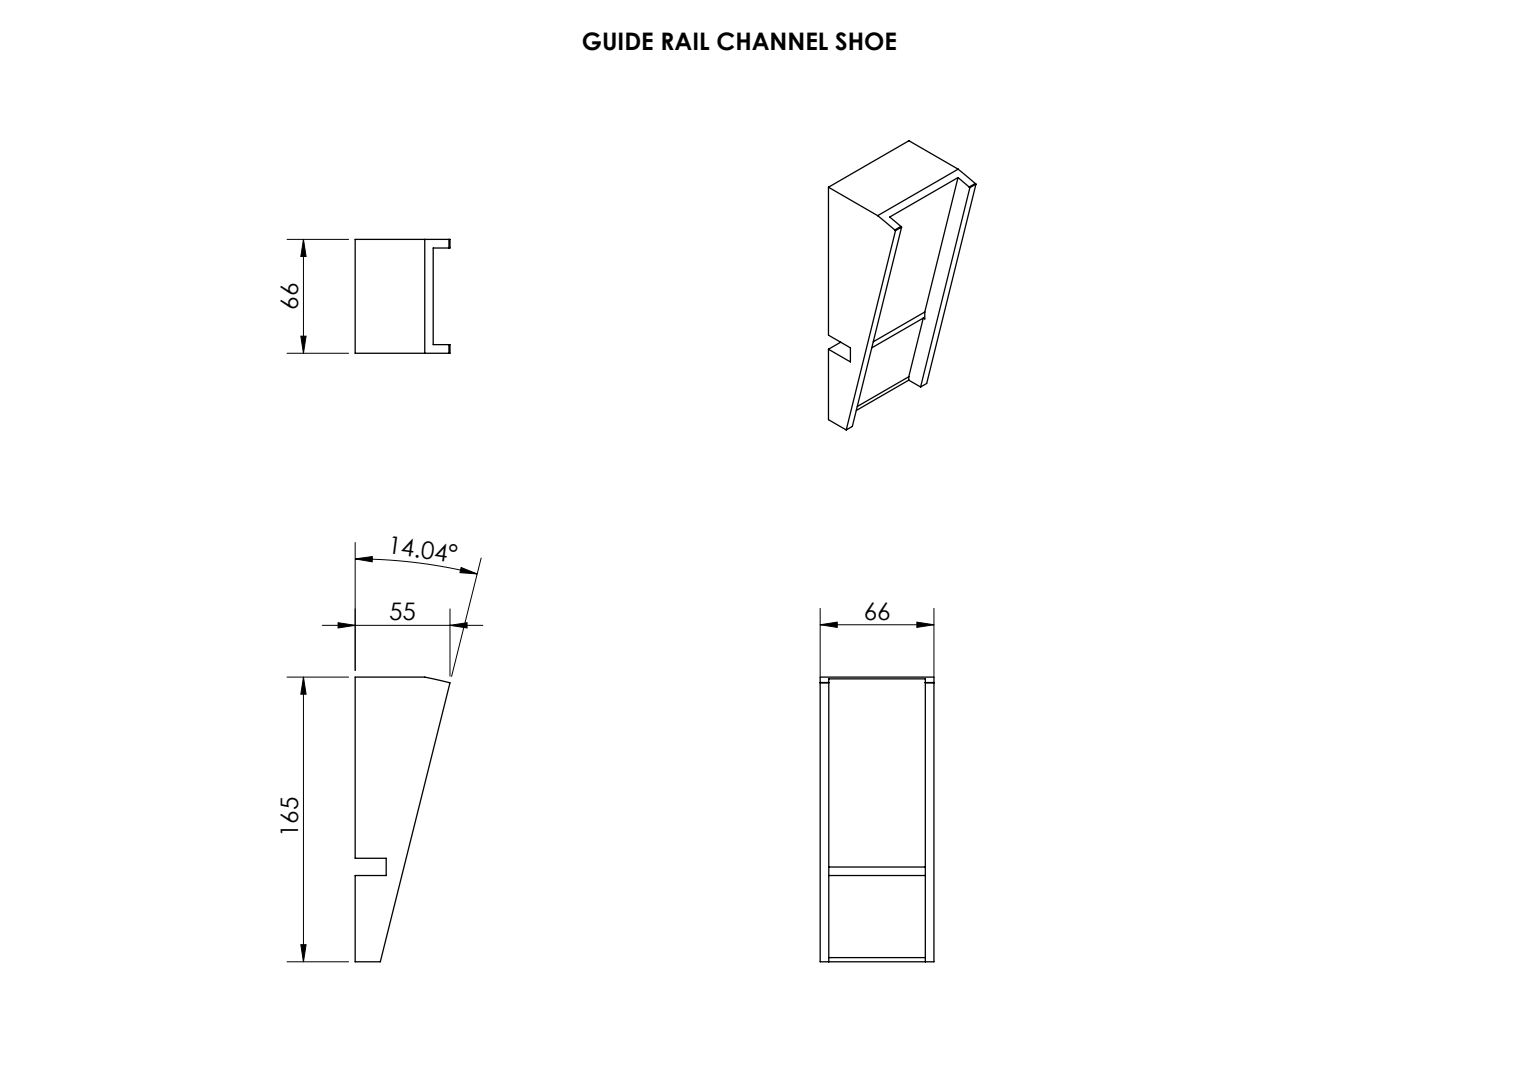
ISO-10303-21;
HEADER;
FILE_DESCRIPTION (('STEP AP214'),
    '1' );
FILE_NAME ('Guide Rail Channel Shoe.step',
    '2026-09-24T10:26:00',
    ( '' ),
    ( '' ),
    'SwSTEP 2.0',
    'SolidWorks 2026',
    '' );
FILE_SCHEMA (( 'AUTOMOTIVE_DESIGN' ));
ENDSEC;

DATA;
#6=CIRCLE ( 'NONE', #8168, 300.0000000000001137 ) ;
#19=DIRECTION ( 'NONE',  ( -0.2425356250363330801, 0.9701425001453319874, 0.000000000000000000 ) ) ;
#29=VERTEX_POINT ( 'NONE', #870 ) ;
#39=LINE ( 'NONE', #7923, #9383 ) ;
#42=( NAMED_UNIT ( * ) SI_UNIT ( $, .STERADIAN. ) SOLID_ANGLE_UNIT ( ) );
#81=ORIENTED_EDGE ( 'NONE', *, *, #3321, .F. ) ;
#100=ORIENTED_EDGE ( 'NONE', *, *, #751, .T. ) ;
#116=DIRECTION ( 'NONE',  ( 1.000000000000000000, 0.000000000000000000, 0.000000000000000000 ) ) ;
#118=EDGE_CURVE ( 'NONE', #4637, #7467, #9051, .T. ) ;
#154=CARTESIAN_POINT ( 'NONE',  ( 58.68170757442803165, 29.57655509336062849, -33.00000000000000000 ) ) ;
#162=DIRECTION ( 'NONE',  ( 0.000000000000000000, -1.000000000000000000, 0.000000000000000000 ) ) ;
#167=CARTESIAN_POINT ( 'NONE',  ( 0.000000000000000000, 0.000000000000000000, 0.000000000000000000 ) ) ;
#169=ORIENTED_EDGE ( 'NONE', *, *, #8329, .T. ) ;
#170=CARTESIAN_POINT ( 'NONE',  ( 59.91362529070399034, 29.57655509336063560, -28.00000000000000000 ) ) ;
#190=EDGE_LOOP ( 'NONE', ( #12989, #13833, #3490, #10771 ) ) ;
#193=PLANE ( 'NONE',  #1641 ) ;
#205=EDGE_CURVE ( 'NONE', #13026, #14419, #660, .T. ) ;
#259=FACE_OUTER_BOUND ( 'NONE', #5577, .T. ) ;
#285=COLOUR_RGB ( '', 0.40784314, 0.44705882, 0.49803922) ;
#310=DIRECTION ( 'NONE',  ( -0.000000000000000000, -0.000000000000000000, -1.000000000000000000 ) ) ;
#325=FILL_AREA_STYLE ('',( #4788 ) ) ;
#345=DIRECTION ( 'NONE',  ( 0.000000000000000000, 0.000000000000000000, -1.000000000000000000 ) ) ;
#366=DIRECTION ( 'NONE',  ( 0.000000000000000000, 0.000000000000000000, 1.000000000000000000 ) ) ;
#390=EDGE_CURVE ( 'NONE', #9890, #13868, #13175, .T. ) ;
#395=DIRECTION ( 'NONE',  ( 1.000000000000000000, 3.916739600140467622E-15, 0.000000000000000000 ) ) ;
#410=VECTOR ( 'NONE', #14385, 1000.000000000000000 ) ;
#431=ORIENTED_EDGE ( 'NONE', *, *, #13902, .F. ) ;
#449=ORIENTED_EDGE ( 'NONE', *, *, #10963, .T. ) ;
#469=CARTESIAN_POINT ( 'NONE',  ( 78.52142056027061301, -86.08568224108226730, -32.99999999999999289 ) ) ;
#487=( GEOMETRIC_REPRESENTATION_CONTEXT ( 3 ) GLOBAL_UNCERTAINTY_ASSIGNED_CONTEXT ( ( #2963 ) ) GLOBAL_UNIT_ASSIGNED_CONTEXT ( ( #1746, #1885, #3068 ) ) REPRESENTATION_CONTEXT ( 'NONE', 'WORKASPACE' ) );
#605=ORIENTED_EDGE ( 'NONE', *, *, #10788, .F. ) ;
#609=DIRECTION ( 'NONE',  ( 0.000000000000000000, -1.000000000000000000, 0.000000000000000000 ) ) ;
#650=LINE ( 'NONE', #12861, #14230 ) ;
#652=FILL_AREA_STYLE_COLOUR ( '', #8179 ) ;
#660=LINE ( 'NONE', #2704, #1726 ) ;
#670=DIRECTION ( 'NONE',  ( -3.916739600140467622E-15, 1.000000000000000000, 0.000000000000000000 ) ) ;
#687=VERTEX_POINT ( 'NONE', #13818 ) ;
#725=DIRECTION ( 'NONE',  ( 0.000000000000000000, -1.000000000000000000, 0.000000000000000000 ) ) ;
#733=DIRECTION ( 'NONE',  ( 0.2425356250363330801, -0.9701425001453319874, -0.000000000000000000 ) ) ;
#748=ORIENTED_EDGE ( 'NONE', *, *, #2973, .T. ) ;
#751=EDGE_CURVE ( 'NONE', #8097, #29, #10582, .T. ) ;
#754=ORIENTED_EDGE ( 'NONE', *, *, #2268, .T. ) ;
#757=ORIENTED_EDGE ( 'NONE', *, *, #2376, .F. ) ;
#758=( GEOMETRIC_REPRESENTATION_CONTEXT ( 3 ) GLOBAL_UNCERTAINTY_ASSIGNED_CONTEXT ( ( #7174 ) ) GLOBAL_UNIT_ASSIGNED_CONTEXT ( ( #1276, #6755, #8134 ) ) REPRESENTATION_CONTEXT ( 'NONE', 'WORKASPACE' ) );
#764=EDGE_LOOP ( 'NONE', ( #5468, #4866, #1029, #12657, #7119, #9076, #4306, #10621 ) ) ;
#774=VECTOR ( 'NONE', #10253, 1000.000000000000000 ) ;
#775=VECTOR ( 'NONE', #609, 1000.000000000000000 ) ;
#798=CARTESIAN_POINT ( 'NONE',  ( 76.68170757442801744, 39.57655509336063204, -33.00000000000000000 ) ) ;
#839=CARTESIAN_POINT ( 'NONE',  ( 31.38313257588132288, 143.6985259526512948, 28.00000000000000000 ) ) ;
#870=CARTESIAN_POINT ( 'NONE',  ( 76.68170757442804586, -20.42344490663941414, 33.00000000000000000 ) ) ;
#917=EDGE_CURVE ( 'NONE', #13885, #9506, #10868, .T. ) ;
#931=PRODUCT_CONTEXT ( 'NONE', #9027, 'mechanical' ) ;
#942=ORIENTED_EDGE ( 'NONE', *, *, #10788, .T. ) ;
#943=PLANE ( 'NONE',  #6123 ) ;
#944=EDGE_CURVE ( 'NONE', #7467, #1783, #14456, .T. ) ;
#954=AXIS2_PLACEMENT_3D ( 'NONE', #1864, #9695, #5154 ) ;
#1023=PRODUCT_DEFINITION_FORMATION_WITH_SPECIFIED_SOURCE ( 'ANY', '', #10212, .NOT_KNOWN. ) ;
#1029=ORIENTED_EDGE ( 'NONE', *, *, #14255, .T. ) ;
#1075=AXIS2_PLACEMENT_3D ( 'NONE', #6445, #8436, #7403 ) ;
#1183=VECTOR ( 'NONE', #14181, 1000.000000000000000 ) ;
#1190=VECTOR ( 'NONE', #3310, 1000.000000000000000 ) ;
#1215=DIRECTION ( 'NONE',  ( -0.2425356250363330801, 0.9701425001453319874, 0.000000000000000000 ) ) ;
#1216=EDGE_LOOP ( 'NONE', ( #3549, #605, #13304, #1795 ) ) ;
#1252=VECTOR ( 'NONE', #1971, 1000.000000000000000 ) ;
#1258=VECTOR ( 'NONE', #5303, 1000.000000000000000 ) ;
#1261=LINE ( 'NONE', #10450, #4207 ) ;
#1268=ORIENTED_EDGE ( 'NONE', *, *, #6526, .F. ) ;
#1276=( LENGTH_UNIT ( ) NAMED_UNIT ( * ) SI_UNIT ( .MILLI., .METRE. ) );
#1286=ORIENTED_EDGE ( 'NONE', *, *, #13904, .T. ) ;
#1342=DIRECTION ( 'NONE',  ( -1.000000000000000000, -1.927470528863119049E-16, 0.000000000000000000 ) ) ;
#1348=FACE_OUTER_BOUND ( 'NONE', #13937, .T. ) ;
#1358=LINE ( 'NONE', #5804, #6464 ) ;
#1366=DIRECTION ( 'NONE',  ( -1.000000000000000000, 0.000000000000000000, 0.000000000000000000 ) ) ;
#1376=CARTESIAN_POINT ( 'NONE',  ( 58.68170757442803165, 29.57655509336062849, -33.00000000000000000 ) ) ;
#1377=VERTEX_POINT ( 'NONE', #1649 ) ;
#1391=LINE ( 'NONE', #7911, #1671 ) ;
#1419=ORIENTED_EDGE ( 'NONE', *, *, #11341, .T. ) ;
#1502=ORIENTED_EDGE ( 'NONE', *, *, #3655, .T. ) ;
#1517=DIRECTION ( 'NONE',  ( 0.000000000000000000, 0.000000000000000000, 1.000000000000000000 ) ) ;
#1531=LINE ( 'NONE', #10681, #1666 ) ;
#1535=EDGE_CURVE ( 'NONE', #11633, #13672, #6590, .T. ) ;
#1586=FACE_OUTER_BOUND ( 'NONE', #7438, .T. ) ;
#1617=EDGE_CURVE ( 'NONE', #6928, #8393, #1391, .T. ) ;
#1637=ORIENTED_EDGE ( 'NONE', *, *, #13104, .T. ) ;
#1641=AXIS2_PLACEMENT_3D ( 'NONE', #5730, #345, #9335 ) ;
#1649=CARTESIAN_POINT ( 'NONE',  ( 22.28098402457126426, 141.4229888148237535, 33.00000000000000000 ) ) ;
#1664=CARTESIAN_POINT ( 'NONE',  ( 95.04167153547044222, -149.6197612287760705, 33.00000000000000000 ) ) ;
#1666=VECTOR ( 'NONE', #5975, 1000.000000000000000 ) ;
#1669=CARTESIAN_POINT ( 'NONE',  ( 76.68170757442804586, -20.42344490663941414, -33.00000000000000000 ) ) ;
#1671=VECTOR ( 'NONE', #310, 1000.000000000000000 ) ;
#1726=VECTOR ( 'NONE', #12961, 1000.000000000000000 ) ;
#1737=FACE_OUTER_BOUND ( 'NONE', #5106, .T. ) ;
#1746=( LENGTH_UNIT ( ) NAMED_UNIT ( * ) SI_UNIT ( .MILLI., .METRE. ) );
#1767=VERTEX_POINT ( 'NONE', #4988 ) ;
#1780=CARTESIAN_POINT ( 'NONE',  ( 78.52142056027061301, -86.08568224108226730, 28.00000000000000000 ) ) ;
#1783=VERTEX_POINT ( 'NONE', #7388 ) ;
#1784=UNCERTAINTY_MEASURE_WITH_UNIT (LENGTH_MEASURE( 1.000000000000000082E-05 ), #2241, 'distance_accuracy_value', 'NONE');
#1795=ORIENTED_EDGE ( 'NONE', *, *, #3657, .T. ) ;
#1814=ORIENTED_EDGE ( 'NONE', *, *, #7517, .T. ) ;
#1859=FACE_OUTER_BOUND ( 'NONE', #4265, .T. ) ;
#1863=ORIENTED_EDGE ( 'NONE', *, *, #8702, .F. ) ;
#1864=CARTESIAN_POINT ( 'NONE',  ( 36.31750732272606541, 144.5765550933605823, -199.4258611313499330 ) ) ;
#1885=( NAMED_UNIT ( * ) PLANE_ANGLE_UNIT ( ) SI_UNIT ( $, .RADIAN. ) );
#1923=AXIS2_PLACEMENT_3D ( 'NONE', #4562, #13481, #7898 ) ;
#1971=DIRECTION ( 'NONE',  ( 1.000000000000000000, 1.927470528863119049E-16, 0.000000000000000000 ) ) ;
#1973=PLANE ( 'NONE',  #10047 ) ;
#1995=DIRECTION ( 'NONE',  ( 1.000000000000000000, 0.000000000000000000, -3.576224061345501491E-16 ) ) ;
#2002=DIRECTION ( 'NONE',  ( -0.000000000000000000, -0.000000000000000000, -1.000000000000000000 ) ) ;
#2034=DIRECTION ( 'NONE',  ( 0.000000000000000000, 0.000000000000000000, -1.000000000000000000 ) ) ;
#2035=PLANE ( 'NONE',  #4449 ) ;
#2041=DIRECTION ( 'NONE',  ( 0.9701425001453325425, 0.2425356250363304988, 0.000000000000000000 ) ) ;
#2052=CARTESIAN_POINT ( 'NONE',  ( 71.80728622811317052, -20.42344490663941414, -27.99999999999999645 ) ) ;
#2080=ORIENTED_EDGE ( 'NONE', *, *, #12073, .T. ) ;
#2089=LINE ( 'NONE', #6752, #7978 ) ;
#2103=ORIENTED_EDGE ( 'NONE', *, *, #3418, .F. ) ;
#2109=FACE_OUTER_BOUND ( 'NONE', #10942, .T. ) ;
#2143=DIRECTION ( 'NONE',  ( 0.9701425001453319874, 0.2425356250363330801, 0.000000000000000000 ) ) ;
#2160=LINE ( 'NONE', #9912, #410 ) ;
#2164=AXIS2_PLACEMENT_3D ( 'NONE', #9423, #13830, #1366 ) ;
#2170=CARTESIAN_POINT ( 'NONE',  ( 59.91362529070399034, 29.57655509336062849, -28.00000000000000000 ) ) ;
#2171=DIRECTION ( 'NONE',  ( -3.916739600140467622E-15, 1.000000000000000000, 0.000000000000000000 ) ) ;
#2188=ORIENTED_EDGE ( 'NONE', *, *, #3988, .F. ) ;
#2219=CARTESIAN_POINT ( 'NONE',  ( 0.000000000000000000, -20.42344490663941414, -33.00000000000000000 ) ) ;
#2241=( LENGTH_UNIT ( ) NAMED_UNIT ( * ) SI_UNIT ( .MILLI., .METRE. ) );
#2245=ORIENTED_EDGE ( 'NONE', *, *, #6820, .F. ) ;
#2253=ADVANCED_FACE ( 'NONE', ( #2109 ), #2035, .F. ) ;
#2268=EDGE_CURVE ( 'NONE', #9459, #1783, #14266, .T. ) ;
#2272=FACE_OUTER_BOUND ( 'NONE', #2925, .T. ) ;
#2280=DIRECTION ( 'NONE',  ( -1.000000000000000000, 0.000000000000000000, 0.000000000000000000 ) ) ;
#2283=DIRECTION ( 'NONE',  ( -0.000000000000000000, -0.000000000000000000, -1.000000000000000000 ) ) ;
#2299=ORIENTED_EDGE ( 'NONE', *, *, #1535, .F. ) ;
#2316=VERTEX_POINT ( 'NONE', #8252 ) ;
#2362=VECTOR ( 'NONE', #9044, 1000.000000000000000 ) ;
#2367=VECTOR ( 'NONE', #2283, 1000.000000000000000 ) ;
#2376=EDGE_CURVE ( 'NONE', #9459, #11964, #1358, .T. ) ;
#2471=LINE ( 'NONE', #13614, #2362 ) ;
#2591=DIRECTION ( 'NONE',  ( 0.000000000000000000, 0.000000000000000000, 1.000000000000000000 ) ) ;
#2624=MECHANICAL_DESIGN_GEOMETRIC_PRESENTATION_REPRESENTATION('',(#10328),#11983);
#2671=CARTESIAN_POINT ( 'NONE',  ( 71.80728622811317052, -17.99808865627608512, -28.00000000000000000 ) ) ;
#2688=CARTESIAN_POINT ( 'NONE',  ( 76.68170757442804586, -20.42344490663941414, -199.4258611313499330 ) ) ;
#2691=ADVANCED_FACE ( 'NONE', ( #14116 ), #6465, .T. ) ;
#2692=FACE_OUTER_BOUND ( 'NONE', #4554, .T. ) ;
#2704=CARTESIAN_POINT ( 'NONE',  ( 76.68170757442801744, 144.5765550933605823, -199.4258611313499330 ) ) ;
#2837=VECTOR ( 'NONE', #366, 1000.000000000000000 ) ;
#2894=ORIENTED_EDGE ( 'NONE', *, *, #12073, .F. ) ;
#2925=EDGE_LOOP ( 'NONE', ( #10674, #14163, #9249, #8632, #13072, #942, #12028, #2103 ) ) ;
#2951=ORIENTED_EDGE ( 'NONE', *, *, #2973, .F. ) ;
#2958=VECTOR ( 'NONE', #3985, 999.9999999999998863 ) ;
#2963=UNCERTAINTY_MEASURE_WITH_UNIT (LENGTH_MEASURE( 1.000000000000000082E-05 ), #1746, 'distance_accuracy_value', 'NONE');
#2969=PLANE ( 'NONE',  #1075 ) ;
#2973=EDGE_CURVE ( 'NONE', #5297, #4637, #12601, .T. ) ;
#2992=DIRECTION ( 'NONE',  ( 1.000000000000000000, 3.916739600140467622E-15, 0.000000000000000000 ) ) ;
#3010=DIRECTION ( 'NONE',  ( -0.9701425001453325425, -0.2425356250363304988, 0.000000000000000000 ) ) ;
#3011=CARTESIAN_POINT ( 'NONE',  ( 62.10586122665989706, -20.42344490663939993, 33.00000000000000000 ) ) ;
#3060=DIRECTION ( 'NONE',  ( 1.000000000000000000, 0.000000000000000000, 0.000000000000000000 ) ) ;
#3068=( NAMED_UNIT ( * ) SI_UNIT ( $, .STERADIAN. ) SOLID_ANGLE_UNIT ( ) );
#3120=CARTESIAN_POINT ( 'NONE',  ( 88.22284556172391490, -83.66032599071898801, -28.00000000000000000 ) ) ;
#3144=EDGE_CURVE ( 'NONE', #5297, #4481, #12833, .T. ) ;
#3174=LINE ( 'NONE', #2219, #6591 ) ;
#3310=DIRECTION ( 'NONE',  ( 1.000000000000000000, 0.000000000000000000, 0.000000000000000000 ) ) ;
#3318=VECTOR ( 'NONE', #670, 1000.000000000000000 ) ;
#3321=EDGE_CURVE ( 'NONE', #6195, #10355, #8937, .T. ) ;
#3340=CARTESIAN_POINT ( 'NONE',  ( 22.28098402457129268, 141.4229888148237251, 28.00000000000000000 ) ) ;
#3343=ORIENTED_EDGE ( 'NONE', *, *, #944, .F. ) ;
#3345=DIRECTION ( 'NONE',  ( 0.000000000000000000, 0.000000000000000000, 1.000000000000000000 ) ) ;
#3359=ORIENTED_EDGE ( 'NONE', *, *, #5495, .T. ) ;
#3402=EDGE_CURVE ( 'NONE', #13672, #4341, #11854, .T. ) ;
#3418=EDGE_CURVE ( 'NONE', #1767, #6248, #10583, .T. ) ;
#3448=DIRECTION ( 'NONE',  ( -1.000000000000000000, 0.000000000000000000, 0.000000000000000000 ) ) ;
#3487=( NAMED_UNIT ( * ) PLANE_ANGLE_UNIT ( ) SI_UNIT ( $, .RADIAN. ) );
#3490=ORIENTED_EDGE ( 'NONE', *, *, #5495, .F. ) ;
#3533=VECTOR ( 'NONE', #10987, 1000.000000000000000 ) ;
#3541=ADVANCED_FACE ( 'NONE', ( #1737 ), #9841, .T. ) ;
#3542=VECTOR ( 'NONE', #3817, 1000.000000000000000 ) ;
#3549=ORIENTED_EDGE ( 'NONE', *, *, #9120, .T. ) ;
#3622=EDGE_CURVE ( 'NONE', #6997, #10870, #2089, .T. ) ;
#3627=CARTESIAN_POINT ( 'NONE',  ( 76.68170757442796059, 3.003422806631532356E-13, -199.4258611313499330 ) ) ;
#3638=CIRCLE ( 'NONE', #12999, 300.0000000000001137 ) ;
#3642=VERTEX_POINT ( 'NONE', #8877 ) ;
#3655=EDGE_CURVE ( 'NONE', #4481, #7467, #6833, .T. ) ;
#3657=EDGE_CURVE ( 'NONE', #5508, #3642, #39, .T. ) ;
#3662=LINE ( 'NONE', #8098, #8406 ) ;
#3722=LINE ( 'NONE', #6781, #7013 ) ;
#3757=LINE ( 'NONE', #11573, #12946 ) ;
#3817=DIRECTION ( 'NONE',  ( -1.000000000000000000, 0.000000000000000000, 0.000000000000000000 ) ) ;
#3901=EDGE_CURVE ( 'NONE', #4341, #6772, #14016, .T. ) ;
#3912=FACE_OUTER_BOUND ( 'NONE', #190, .T. ) ;
#3916=VECTOR ( 'NONE', #1215, 999.9999999999998863 ) ;
#3981=AXIS2_PLACEMENT_3D ( 'NONE', #8549, #9580, #3010 ) ;
#3985=DIRECTION ( 'NONE',  ( -0.9701425001453319874, -0.2425356250363330801, -0.000000000000000000 ) ) ;
#3988=EDGE_CURVE ( 'NONE', #1377, #11964, #7544, .T. ) ;
#4054=CARTESIAN_POINT ( 'NONE',  ( 58.68170757442803165, -86.08568224108226730, -28.00000000000000000 ) ) ;
#4068=ORIENTED_EDGE ( 'NONE', *, *, #10686, .T. ) ;
#4128=VERTEX_POINT ( 'NONE', #14373 ) ;
#4158=ORIENTED_EDGE ( 'NONE', *, *, #12918, .T. ) ;
#4207=VECTOR ( 'NONE', #162, 1000.000000000000000 ) ;
#4265=EDGE_LOOP ( 'NONE', ( #2188, #13222, #7506, #10107 ) ) ;
#4270=VECTOR ( 'NONE', #8995, 999.9999999999998863 ) ;
#4306=ORIENTED_EDGE ( 'NONE', *, *, #390, .T. ) ;
#4319=CARTESIAN_POINT ( 'NONE',  ( 88.22284556172391490, -83.66032599071898801, 28.00000000000000000 ) ) ;
#4341=VERTEX_POINT ( 'NONE', #11796 ) ;
#4345=CARTESIAN_POINT ( 'NONE',  ( 36.31750732272606541, 144.5765550933605823, 33.00000000000000000 ) ) ;
#4352=EDGE_CURVE ( 'NONE', #13229, #9890, #8564, .T. ) ;
#4353=FACE_OUTER_BOUND ( 'NONE', #9545, .T. ) ;
#4361=EDGE_CURVE ( 'NONE', #1377, #13885, #6147, .T. ) ;
#4362=CARTESIAN_POINT ( 'NONE',  ( 58.68170757442803165, 29.57655509336062849, -28.00000000000000000 ) ) ;
#4387=ORIENTED_EDGE ( 'NONE', *, *, #944, .T. ) ;
#4437=LINE ( 'NONE', #8794, #3533 ) ;
#4449=AXIS2_PLACEMENT_3D ( 'NONE', #5324, #13310, #8550 ) ;
#4481=VERTEX_POINT ( 'NONE', #2052 ) ;
#4483=VECTOR ( 'NONE', #1342, 1000.000000000000000 ) ;
#4488=ADVANCED_FACE ( 'NONE', ( #2272 ), #943, .F. ) ;
#4536=ORIENTED_EDGE ( 'NONE', *, *, #9120, .F. ) ;
#4554=EDGE_LOOP ( 'NONE', ( #11599, #8685, #6383, #1863, #11350, #2894, #13470, #4387, #4158 ) ) ;
#4561=ADVANCED_BREP_SHAPE_REPRESENTATION ( '', ( #11635, #11025 ), #758 ) ;
#4562=CARTESIAN_POINT ( 'NONE',  ( 76.68170757442801744, 29.57655509336063204, -33.00000000000000000 ) ) ;
#4618=CARTESIAN_POINT ( 'NONE',  ( 58.68170757442803165, 39.57655509336063204, -33.00000000000000000 ) ) ;
#4637=VERTEX_POINT ( 'NONE', #7003 ) ;
#4640=EDGE_LOOP ( 'NONE', ( #8368, #1419, #13334, #100, #2245, #754, #3343, #7325 ) ) ;
#4644=VECTOR ( 'NONE', #12554, 1000.000000000000000 ) ;
#4655=ORIENTED_EDGE ( 'NONE', *, *, #3657, .F. ) ;
#4719=SURFACE_SIDE_STYLE ('',( #12473 ) ) ;
#4731=VERTEX_POINT ( 'NONE', #7629 ) ;
#4732=CARTESIAN_POINT ( 'NONE',  ( 31.41872415839353039, 143.5561596226025074, -28.00000000000000000 ) ) ;
#4733=ORIENTED_EDGE ( 'NONE', *, *, #10431, .F. ) ;
#4734=ORIENTED_EDGE ( 'NONE', *, *, #390, .F. ) ;
#4744=ORIENTED_EDGE ( 'NONE', *, *, #1617, .T. ) ;
#4788=FILL_AREA_STYLE_COLOUR ( '', #285 ) ;
#4831=VECTOR ( 'NONE', #11737, 1000.000000000000000 ) ;
#4832=EDGE_LOOP ( 'NONE', ( #9169, #12336, #14242, #4068 ) ) ;
#4866=ORIENTED_EDGE ( 'NONE', *, *, #3418, .T. ) ;
#4918=CARTESIAN_POINT ( 'NONE',  ( 21.68170757442799967, 141.2731697022880155, -28.00000000000000000 ) ) ;
#4934=CARTESIAN_POINT ( 'NONE',  ( 21.68170757442799967, 141.2731697022880155, -32.99999999999999289 ) ) ;
#4951=AXIS2_PLACEMENT_3D ( 'NONE', #10869, #8532, #3060 ) ;
#4953=EDGE_CURVE ( 'NONE', #13868, #9429, #7712, .T. ) ;
#4985=ORIENTED_EDGE ( 'NONE', *, *, #205, .T. ) ;
#4988=CARTESIAN_POINT ( 'NONE',  ( 58.68170757442803165, 29.57655509336062849, 27.99999999999999645 ) ) ;
#5026=LINE ( 'NONE', #5170, #1183 ) ;
#5027=EDGE_CURVE ( 'NONE', #8393, #11633, #3638, .T. ) ;
#5055=DIRECTION ( 'NONE',  ( -0.000000000000000000, -0.000000000000000000, -1.000000000000000000 ) ) ;
#5082=ADVANCED_FACE ( 'NONE', ( #3912 ), #8061, .T. ) ;
#5104=ORIENTED_EDGE ( 'NONE', *, *, #2376, .T. ) ;
#5106=EDGE_LOOP ( 'NONE', ( #11663, #6184, #10149, #7042, #11543, #2299, #7476, #9228 ) ) ;
#5135=DIRECTION ( 'NONE',  ( -0.2425356250363330801, 0.9701425001453319874, 0.000000000000000000 ) ) ;
#5145=ORIENTED_EDGE ( 'NONE', *, *, #6298, .T. ) ;
#5154=DIRECTION ( 'NONE',  ( 0.000000000000000000, 0.000000000000000000, -1.000000000000000000 ) ) ;
#5170=CARTESIAN_POINT ( 'NONE',  ( 76.68170757442801744, 39.57655509336063204, -33.00000000000000000 ) ) ;
#5172=ADVANCED_FACE ( 'NONE', ( #1859 ), #2969, .F. ) ;
#5190=LINE ( 'NONE', #12970, #9623 ) ;
#5195=VECTOR ( 'NONE', #11598, 1000.000000000000000 ) ;
#5292=EDGE_LOOP ( 'NONE', ( #12843, #7817, #748, #2080 ) ) ;
#5294=LINE ( 'NONE', #3120, #12559 ) ;
#5295=EDGE_CURVE ( 'NONE', #13026, #5508, #3662, .T. ) ;
#5297=VERTEX_POINT ( 'NONE', #11472 ) ;
#5303=DIRECTION ( 'NONE',  ( -0.9701425001453325425, -0.2425356250363304988, 0.000000000000000000 ) ) ;
#5323=CARTESIAN_POINT ( 'NONE',  ( 76.68170757442796059, 3.003422806631532356E-13, 33.00000000000000000 ) ) ;
#5324=CARTESIAN_POINT ( 'NONE',  ( 78.52142056027061301, -86.08568224108226730, -28.00000000000000000 ) ) ;
#5391=CARTESIAN_POINT ( 'NONE',  ( 78.52142056027055617, 29.57655509336062849, -28.00000000000000000 ) ) ;
#5417=PLANE ( 'NONE',  #1923 ) ;
#5429=ADVANCED_FACE ( 'NONE', ( #8481 ), #7374, .F. ) ;
#5441=DIRECTION ( 'NONE',  ( 1.000000000000000000, 0.000000000000000000, 0.000000000000000000 ) ) ;
#5466=EDGE_CURVE ( 'NONE', #13885, #6928, #6, .T. ) ;
#5468=ORIENTED_EDGE ( 'NONE', *, *, #11730, .T. ) ;
#5492=LINE ( 'NONE', #9961, #4270 ) ;
#5495=EDGE_CURVE ( 'NONE', #29, #687, #7507, .T. ) ;
#5498=PLANE ( 'NONE',  #13650 ) ;
#5500=ADVANCED_FACE ( 'NONE', ( #13102 ), #1973, .T. ) ;
#5507=ORIENTED_EDGE ( 'NONE', *, *, #5027, .T. ) ;
#5508=VERTEX_POINT ( 'NONE', #798 ) ;
#5518=CARTESIAN_POINT ( 'NONE',  ( 71.80728622811317052, -20.42344490663941414, 28.00000000000000000 ) ) ;
#5528=AXIS2_PLACEMENT_3D ( 'NONE', #12031, #2002, #13351 ) ;
#5538=LINE ( 'NONE', #10010, #6079 ) ;
#5577=EDGE_LOOP ( 'NONE', ( #1286, #5507, #8075, #7936, #12667, #10442, #1814, #4734, #12975 ) ) ;
#5635=CARTESIAN_POINT ( 'NONE',  ( 22.28098402457126426, 141.4229888148238103, 1.219362754841566419E-12 ) ) ;
#5653=FACE_OUTER_BOUND ( 'NONE', #8593, .T. ) ;
#5654=CARTESIAN_POINT ( 'NONE',  ( 95.04167153547044222, -149.6197612287760705, -28.00000000000000000 ) ) ;
#5694=LINE ( 'NONE', #154, #9376 ) ;
#5730=CARTESIAN_POINT ( 'NONE',  ( 88.22284556172391490, -83.66032599071898801, 28.00000000000000000 ) ) ;
#5768=ADVANCED_FACE ( 'NONE', ( #2692 ), #193, .T. ) ;
#5793=ORIENTED_EDGE ( 'NONE', *, *, #3321, .T. ) ;
#5794=PLANE ( 'NONE',  #11865 ) ;
#5804=CARTESIAN_POINT ( 'NONE',  ( 78.52142056027061301, -86.08568224108226730, 33.00000000000000000 ) ) ;
#5849=EDGE_CURVE ( 'NONE', #5508, #6997, #5026, .T. ) ;
#5870=DIRECTION ( 'NONE',  ( 1.000000000000000000, 0.000000000000000000, 0.000000000000000000 ) ) ;
#5886=LINE ( 'NONE', #11384, #4644 ) ;
#5897=ORIENTED_EDGE ( 'NONE', *, *, #3402, .T. ) ;
#5938=CARTESIAN_POINT ( 'NONE',  ( 78.52142056027061301, -86.08568224108226730, -28.00000000000000000 ) ) ;
#5958=CARTESIAN_POINT ( 'NONE',  ( 59.91362529070399034, 29.57655509336062849, 28.00000000000000000 ) ) ;
#5975=DIRECTION ( 'NONE',  ( 0.000000000000000000, 0.000000000000000000, -1.000000000000000000 ) ) ;
#5983=VECTOR ( 'NONE', #2591, 1000.000000000000000 ) ;
#5993=ADVANCED_FACE ( 'NONE', ( #5653 ), #11578, .F. ) ;
#5999=PRODUCT_DEFINITION_SHAPE ( 'NONE', 'NONE',  #12500 ) ;
#6047=ORIENTED_EDGE ( 'NONE', *, *, #5295, .T. ) ;
#6055=LINE ( 'NONE', #13630, #3542 ) ;
#6079=VECTOR ( 'NONE', #2041, 1000.000000000000000 ) ;
#6101=ORIENTED_EDGE ( 'NONE', *, *, #10400, .T. ) ;
#6113=DIRECTION ( 'NONE',  ( -0.000000000000000000, -0.000000000000000000, 1.000000000000000000 ) ) ;
#6123=AXIS2_PLACEMENT_3D ( 'NONE', #10094, #3448, #14356 ) ;
#6139=AXIS2_PLACEMENT_3D ( 'NONE', #7558, #6250, #8449 ) ;
#6146=VECTOR ( 'NONE', #13427, 1000.000000000000000 ) ;
#6147=LINE ( 'NONE', #14214, #11993 ) ;
#6184=ORIENTED_EDGE ( 'NONE', *, *, #4361, .F. ) ;
#6195=VERTEX_POINT ( 'NONE', #10784 ) ;
#6196=CARTESIAN_POINT ( 'NONE',  ( 22.28098402457126426, 141.4229888148238103, -28.00000000000000000 ) ) ;
#6248=VERTEX_POINT ( 'NONE', #14444 ) ;
#6250=DIRECTION ( 'NONE',  ( -0.9701425001453319874, -0.2425356250363330801, 0.000000000000000000 ) ) ;
#6280=LINE ( 'NONE', #9725, #3318 ) ;
#6298=EDGE_CURVE ( 'NONE', #10870, #2316, #4437, .T. ) ;
#6302=ORIENTED_EDGE ( 'NONE', *, *, #10686, .F. ) ;
#6352=DIRECTION ( 'NONE',  ( 0.000000000000000000, 1.000000000000000000, 0.000000000000000000 ) ) ;
#6382=CARTESIAN_POINT ( 'NONE',  ( 71.80728622811317052, 38.49793223363091954, -28.00000000000000000 ) ) ;
#6383=ORIENTED_EDGE ( 'NONE', *, *, #8329, .F. ) ;
#6394=ORIENTED_EDGE ( 'NONE', *, *, #3988, .T. ) ;
#6425=ORIENTED_EDGE ( 'NONE', *, *, #5849, .T. ) ;
#6445=CARTESIAN_POINT ( 'NONE',  ( -31.96535124910143821, 127.8614049964057813, 1.219362754841566419E-12 ) ) ;
#6464=VECTOR ( 'NONE', #12491, 999.9999999999998863 ) ;
#6465=PLANE ( 'NONE',  #14233 ) ;
#6508=CARTESIAN_POINT ( 'NONE',  ( 62.10586122665986863, -20.42344490663941414, -27.99999999999999645 ) ) ;
#6524=DIRECTION ( 'NONE',  ( 0.000000000000000000, 0.000000000000000000, 1.000000000000000000 ) ) ;
#6526=EDGE_CURVE ( 'NONE', #10492, #6248, #1261, .T. ) ;
#6590=LINE ( 'NONE', #5635, #2367 ) ;
#6591=VECTOR ( 'NONE', #2280, 1000.000000000000000 ) ;
#6622=LINE ( 'NONE', #4319, #3916 ) ;
#6659=LINE ( 'NONE', #6508, #8116 ) ;
#6737=LINE ( 'NONE', #14368, #6146 ) ;
#6739=PRODUCT_DEFINITION_CONTEXT ( 'detailed design', #10449, 'design' ) ;
#6752=CARTESIAN_POINT ( 'NONE',  ( 58.68170757442803165, 39.57655509336063204, -33.00000000000000000 ) ) ;
#6755=( NAMED_UNIT ( * ) PLANE_ANGLE_UNIT ( ) SI_UNIT ( $, .RADIAN. ) );
#6772=VERTEX_POINT ( 'NONE', #11602 ) ;
#6781=CARTESIAN_POINT ( 'NONE',  ( 76.68170757442796059, 3.003422806631532356E-13, -33.00000000000000000 ) ) ;
#6789=DIRECTION ( 'NONE',  ( 0.000000000000000000, -1.000000000000000000, 0.000000000000000000 ) ) ;
#6820=EDGE_CURVE ( 'NONE', #9459, #29, #5886, .T. ) ;
#6833=LINE ( 'NONE', #11299, #12432 ) ;
#6928=VERTEX_POINT ( 'NONE', #13411 ) ;
#6990=CARTESIAN_POINT ( 'NONE',  ( 21.68170757442799967, 141.2731697022880155, -32.99999999999999289 ) ) ;
#6997=VERTEX_POINT ( 'NONE', #11092 ) ;
#7003=CARTESIAN_POINT ( 'NONE',  ( 71.80728622811317052, -17.99808865627608512, 28.00000000000000000 ) ) ;
#7011=CARTESIAN_POINT ( 'NONE',  ( 58.68170757442803165, 34.50422595846453078, -28.00000000000000000 ) ) ;
#7013=VECTOR ( 'NONE', #7878, 1000.000000000000000 ) ;
#7042=ORIENTED_EDGE ( 'NONE', *, *, #3901, .F. ) ;
#7119=ORIENTED_EDGE ( 'NONE', *, *, #6298, .F. ) ;
#7121=FACE_OUTER_BOUND ( 'NONE', #7956, .T. ) ;
#7127=DIRECTION ( 'NONE',  ( 0.000000000000000000, 0.000000000000000000, 1.000000000000000000 ) ) ;
#7128=CARTESIAN_POINT ( 'NONE',  ( 58.68170757442803165, 29.57655509336062849, -33.00000000000000000 ) ) ;
#7171=DIRECTION ( 'NONE',  ( -0.2425356250363330801, 0.9701425001453319874, 0.000000000000000000 ) ) ;
#7174=UNCERTAINTY_MEASURE_WITH_UNIT (LENGTH_MEASURE( 1.000000000000000082E-05 ), #1276, 'distance_accuracy_value', 'NONE');
#7190=LINE ( 'NONE', #4934, #10247 ) ;
#7298=EDGE_CURVE ( 'NONE', #10355, #13672, #7190, .T. ) ;
#7304=ORIENTED_EDGE ( 'NONE', *, *, #12918, .F. ) ;
#7310=PLANE ( 'NONE',  #8448 ) ;
#7325=ORIENTED_EDGE ( 'NONE', *, *, #3655, .F. ) ;
#7344=FACE_OUTER_BOUND ( 'NONE', #4832, .T. ) ;
#7374=PLANE ( 'NONE',  #3981 ) ;
#7388=CARTESIAN_POINT ( 'NONE',  ( 62.10586122665986863, -20.42344490663941414, 28.00000000000000000 ) ) ;
#7389=SHAPE_REPRESENTATION ( 'Guide Rail Channel Shoe', ( #11025 ), #758 ) ;
#7403=DIRECTION ( 'NONE',  ( -0.9701425001453325425, -0.2425356250363304988, 0.000000000000000000 ) ) ;
#7413=PLANE ( 'NONE',  #6139 ) ;
#7426=PRESENTATION_STYLE_ASSIGNMENT (( #9639 ) ) ;
#7438=EDGE_LOOP ( 'NONE', ( #6302, #8058, #6394, #757, #11181, #3359, #11732, #1268, #4536, #9883 ) ) ;
#7467=VERTEX_POINT ( 'NONE', #11078 ) ;
#7476=ORIENTED_EDGE ( 'NONE', *, *, #5027, .F. ) ;
#7506=ORIENTED_EDGE ( 'NONE', *, *, #917, .T. ) ;
#7507=LINE ( 'NONE', #5323, #11678 ) ;
#7508=VECTOR ( 'NONE', #5135, 999.9999999999998863 ) ;
#7510=DIRECTION ( 'NONE',  ( 0.000000000000000000, 0.000000000000000000, -1.000000000000000000 ) ) ;
#7512=CARTESIAN_POINT ( 'NONE',  ( 76.68170757442801744, 39.57655509336063204, 33.00000000000000000 ) ) ;
#7513=FACE_OUTER_BOUND ( 'NONE', #1216, .T. ) ;
#7517=EDGE_CURVE ( 'NONE', #5297, #13868, #5294, .T. ) ;
#7544=LINE ( 'NONE', #11810, #2958 ) ;
#7555=VECTOR ( 'NONE', #8056, 1000.000000000000000 ) ;
#7558=CARTESIAN_POINT ( 'NONE',  ( 88.22284556172391490, -83.66032599071898801, -28.00000000000000000 ) ) ;
#7629=CARTESIAN_POINT ( 'NONE',  ( 58.68170757442803165, 34.50422595846454499, 28.00000000000000000 ) ) ;
#7712=LINE ( 'NONE', #2170, #12809 ) ;
#7757=DIRECTION ( 'NONE',  ( 0.000000000000000000, 0.000000000000000000, 1.000000000000000000 ) ) ;
#7817=ORIENTED_EDGE ( 'NONE', *, *, #7517, .F. ) ;
#7843=DIRECTION ( 'NONE',  ( -0.2425356250363330801, 0.9701425001453319874, 0.000000000000000000 ) ) ;
#7846=VERTEX_POINT ( 'NONE', #10772 ) ;
#7878=DIRECTION ( 'NONE',  ( 3.916739600140467622E-15, -1.000000000000000000, -0.000000000000000000 ) ) ;
#7898=DIRECTION ( 'NONE',  ( 1.000000000000000000, 1.927470528863118802E-16, 0.000000000000000000 ) ) ;
#7911=CARTESIAN_POINT ( 'NONE',  ( 31.41872415839353039, 143.5561596226024790, 28.00000000000000000 ) ) ;
#7923=CARTESIAN_POINT ( 'NONE',  ( 76.68170757442801744, 39.57655509336063204, -33.00000000000000000 ) ) ;
#7934=EDGE_CURVE ( 'NONE', #4128, #4481, #6659, .T. ) ;
#7936=ORIENTED_EDGE ( 'NONE', *, *, #9847, .F. ) ;
#7955=CARTESIAN_POINT ( 'NONE',  ( 71.80728622811317052, 38.49793223363091954, 28.00000000000000000 ) ) ;
#7956=EDGE_LOOP ( 'NONE', ( #169, #4744, #12317, #4733 ) ) ;
#7978=VECTOR ( 'NONE', #13374, 1000.000000000000000 ) ;
#8056=DIRECTION ( 'NONE',  ( -1.000000000000000000, 0.000000000000000000, -3.576224061345501491E-16 ) ) ;
#8058=ORIENTED_EDGE ( 'NONE', *, *, #10577, .T. ) ;
#8061=PLANE ( 'NONE',  #10645 ) ;
#8075=ORIENTED_EDGE ( 'NONE', *, *, #10303, .F. ) ;
#8090=ORIENTED_EDGE ( 'NONE', *, *, #2268, .F. ) ;
#8097=VERTEX_POINT ( 'NONE', #1669 ) ;
#8098=CARTESIAN_POINT ( 'NONE',  ( 76.68170757442796059, 3.003422806631532356E-13, -33.00000000000000000 ) ) ;
#8116=VECTOR ( 'NONE', #1995, 1000.000000000000000 ) ;
#8134=( NAMED_UNIT ( * ) SI_UNIT ( $, .STERADIAN. ) SOLID_ANGLE_UNIT ( ) );
#8168=AXIS2_PLACEMENT_3D ( 'NONE', #10749, #12064, #11850 ) ;
#8179=COLOUR_RGB ( '', 0.40784314, 0.44705882, 0.49803922) ;
#8189=ORIENTED_EDGE ( 'NONE', *, *, #9847, .T. ) ;
#8190=CIRCLE ( 'NONE', #13356, 300.0000000000001137 ) ;
#8220=ORIENTED_EDGE ( 'NONE', *, *, #11206, .F. ) ;
#8252=CARTESIAN_POINT ( 'NONE',  ( 76.68170757442801744, 29.57655509336063204, -33.00000000000000000 ) ) ;
#8290=DIRECTION ( 'NONE',  ( 0.000000000000000000, 0.000000000000000000, 1.000000000000000000 ) ) ;
#8329=EDGE_CURVE ( 'NONE', #4731, #6928, #6622, .T. ) ;
#8351=CARTESIAN_POINT ( 'NONE',  ( 36.31750732272606541, 144.5765550933605823, -199.4258611313499330 ) ) ;
#8357=DIRECTION ( 'NONE',  ( -3.916739600140467622E-15, 1.000000000000000000, 0.000000000000000000 ) ) ;
#8367=DIRECTION ( 'NONE',  ( 1.000000000000000000, 0.000000000000000000, 0.000000000000000000 ) ) ;
#8368=ORIENTED_EDGE ( 'NONE', *, *, #7934, .F. ) ;
#8393=VERTEX_POINT ( 'NONE', #4732 ) ;
#8401=DIRECTION ( 'NONE',  ( 0.000000000000000000, 0.000000000000000000, -1.000000000000000000 ) ) ;
#8406=VECTOR ( 'NONE', #13626, 1000.000000000000000 ) ;
#8436=DIRECTION ( 'NONE',  ( 0.2425356250363304988, -0.9701425001453325425, -0.000000000000000000 ) ) ;
#8448=AXIS2_PLACEMENT_3D ( 'NONE', #12001, #6352, #10829 ) ;
#8449=DIRECTION ( 'NONE',  ( 0.2425356250363330801, -0.9701425001453319874, -0.000000000000000000 ) ) ;
#8475=ADVANCED_FACE ( 'NONE', ( #1348 ), #5794, .F. ) ;
#8481=FACE_OUTER_BOUND ( 'NONE', #11329, .T. ) ;
#8532=DIRECTION ( 'NONE',  ( 0.000000000000000000, 0.000000000000000000, 1.000000000000000000 ) ) ;
#8549=CARTESIAN_POINT ( 'NONE',  ( -31.96535124910143821, 127.8614049964057813, 1.219362754841566419E-12 ) ) ;
#8550=DIRECTION ( 'NONE',  ( -0.2425356250363330801, 0.9701425001453319874, 0.000000000000000000 ) ) ;
#8564=LINE ( 'NONE', #4054, #775 ) ;
#8593=EDGE_LOOP ( 'NONE', ( #12591, #5897, #12415, #6047, #6425, #12852, #5145, #6101, #1637, #5793 ) ) ;
#8632=ORIENTED_EDGE ( 'NONE', *, *, #11989, .F. ) ;
#8685=ORIENTED_EDGE ( 'NONE', *, *, #5466, .T. ) ;
#8702=EDGE_CURVE ( 'NONE', #1767, #4731, #2160, .T. ) ;
#8788=CARTESIAN_POINT ( 'NONE',  ( 78.52142056027061301, -86.08568224108226730, 33.00000000000000000 ) ) ;
#8794=CARTESIAN_POINT ( 'NONE',  ( 76.68170757442801744, 29.57655509336063204, -33.00000000000000000 ) ) ;
#8877=CARTESIAN_POINT ( 'NONE',  ( 76.68170757442801744, 39.57655509336063204, 33.00000000000000000 ) ) ;
#8903=LINE ( 'NONE', #7512, #13753 ) ;
#8937=LINE ( 'NONE', #9820, #12531 ) ;
#8995=DIRECTION ( 'NONE',  ( -0.2425356250363330801, 0.9701425001453319874, 0.000000000000000000 ) ) ;
#9000=ORIENTED_EDGE ( 'NONE', *, *, #7298, .F. ) ;
#9027=APPLICATION_CONTEXT ( 'automotive_design' ) ;
#9044=DIRECTION ( 'NONE',  ( 0.000000000000000000, 0.000000000000000000, -1.000000000000000000 ) ) ;
#9051=LINE ( 'NONE', #7955, #12466 ) ;
#9076=ORIENTED_EDGE ( 'NONE', *, *, #11989, .T. ) ;
#9120=EDGE_CURVE ( 'NONE', #3642, #10492, #8903, .T. ) ;
#9148=AXIS2_PLACEMENT_3D ( 'NONE', #9173, #8290, #8367 ) ;
#9152=ORIENTED_EDGE ( 'NONE', *, *, #5295, .F. ) ;
#9169=ORIENTED_EDGE ( 'NONE', *, *, #205, .F. ) ;
#9173=CARTESIAN_POINT ( 'NONE',  ( 78.52142056027061301, -86.08568224108226730, -28.00000000000000000 ) ) ;
#9228=ORIENTED_EDGE ( 'NONE', *, *, #1617, .F. ) ;
#9239=DIRECTION ( 'NONE',  ( 0.000000000000000000, 0.000000000000000000, 1.000000000000000000 ) ) ;
#9248=PLANE ( 'NONE',  #9148 ) ;
#9249=ORIENTED_EDGE ( 'NONE', *, *, #4352, .T. ) ;
#9313=DIRECTION ( 'NONE',  ( 1.000000000000000000, 0.000000000000000000, 0.000000000000000000 ) ) ;
#9319=CARTESIAN_POINT ( 'NONE',  ( 88.22284556172388648, 29.57655509336062849, 28.00000000000000000 ) ) ;
#9335=DIRECTION ( 'NONE',  ( -1.000000000000000000, 0.000000000000000000, 0.000000000000000000 ) ) ;
#9376=VECTOR ( 'NONE', #7757, 1000.000000000000000 ) ;
#9383=VECTOR ( 'NONE', #3345, 1000.000000000000000 ) ;
#9421=EDGE_CURVE ( 'NONE', #2316, #687, #650, .T. ) ;
#9423=CARTESIAN_POINT ( 'NONE',  ( 88.22284556172391490, -83.66032599071898801, 33.00000000000000000 ) ) ;
#9429=VERTEX_POINT ( 'NONE', #5958 ) ;
#9459=VERTEX_POINT ( 'NONE', #11910 ) ;
#9475=PLANE ( 'NONE',  #954 ) ;
#9495=SURFACE_STYLE_FILL_AREA ( #10668 ) ;
#9496=CARTESIAN_POINT ( 'NONE',  ( 58.68170757442803165, 39.57655509336063915, 33.00000000000000000 ) ) ;
#9506=VERTEX_POINT ( 'NONE', #12118 ) ;
#9545=EDGE_LOOP ( 'NONE', ( #8090, #5104, #449, #7304 ) ) ;
#9580=DIRECTION ( 'NONE',  ( 0.2425356250363304988, -0.9701425001453325425, -0.000000000000000000 ) ) ;
#9585=SHAPE_DEFINITION_REPRESENTATION ( #5999, #7389 ) ;
#9620=CARTESIAN_POINT ( 'NONE',  ( 76.68170757442801744, 144.5765550933605823, 33.00000000000000000 ) ) ;
#9623=VECTOR ( 'NONE', #8401, 1000.000000000000000 ) ;
#9639=SURFACE_STYLE_USAGE ( .BOTH. , #11839 ) ;
#9695=DIRECTION ( 'NONE',  ( 0.000000000000000000, -1.000000000000000000, 0.000000000000000000 ) ) ;
#9725=CARTESIAN_POINT ( 'NONE',  ( 76.68170757442796059, 3.003422806631532356E-13, 33.00000000000000000 ) ) ;
#9820=CARTESIAN_POINT ( 'NONE',  ( 78.52142056027061301, -86.08568224108226730, -32.99999999999999289 ) ) ;
#9841=CYLINDRICAL_SURFACE ( 'NONE', #4951, 300.0000000000001137 ) ;
#9847=EDGE_CURVE ( 'NONE', #4128, #7846, #11743, .T. ) ;
#9883=ORIENTED_EDGE ( 'NONE', *, *, #11206, .T. ) ;
#9890=VERTEX_POINT ( 'NONE', #4362 ) ;
#9912=CARTESIAN_POINT ( 'NONE',  ( 58.68170757442803165, -83.66032599071898801, 28.00000000000000000 ) ) ;
#9955=LINE ( 'NONE', #4345, #1190 ) ;
#9961=CARTESIAN_POINT ( 'NONE',  ( 88.22284556172391490, -83.66032599071898801, 28.00000000000000000 ) ) ;
#9983=VECTOR ( 'NONE', #12832, 1000.000000000000000 ) ;
#10010=CARTESIAN_POINT ( 'NONE',  ( 21.68170757442799967, 141.2731697022880155, -28.00000000000000000 ) ) ;
#10047=AXIS2_PLACEMENT_3D ( 'NONE', #11997, #725, #2034 ) ;
#10094=CARTESIAN_POINT ( 'NONE',  ( 58.68170757442803165, 39.57655509336063204, -33.00000000000000000 ) ) ;
#10107=ORIENTED_EDGE ( 'NONE', *, *, #10963, .F. ) ;
#10131=DIRECTION ( 'NONE',  ( 0.000000000000000000, 0.000000000000000000, 1.000000000000000000 ) ) ;
#10149=ORIENTED_EDGE ( 'NONE', *, *, #10577, .F. ) ;
#10161=ADVANCED_FACE ( 'NONE', ( #10831 ), #11787, .T. ) ;
#10212=PRODUCT ( 'Guide Rail Channel Shoe', 'Guide Rail Channel Shoe', '', ( #931 ) ) ;
#10247=VECTOR ( 'NONE', #13003, 999.9999999999998863 ) ;
#10253=DIRECTION ( 'NONE',  ( 0.000000000000000000, 0.000000000000000000, -1.000000000000000000 ) ) ;
#10273=CARTESIAN_POINT ( 'NONE',  ( 71.80728622811317052, 38.49793223363091954, -28.00000000000000000 ) ) ;
#10303=EDGE_CURVE ( 'NONE', #7846, #11633, #5538, .T. ) ;
#10328=STYLED_ITEM ( 'NONE', ( #11226 ), #4561 ) ;
#10330=VECTOR ( 'NONE', #11513, 999.9999999999998863 ) ;
#10355=VERTEX_POINT ( 'NONE', #6990 ) ;
#10356=DIRECTION ( 'NONE',  ( 0.000000000000000000, 0.000000000000000000, -1.000000000000000000 ) ) ;
#10359=ORIENTED_EDGE ( 'NONE', *, *, #118, .F. ) ;
#10400=EDGE_CURVE ( 'NONE', #2316, #8097, #3722, .T. ) ;
#10431=EDGE_CURVE ( 'NONE', #4731, #13229, #2471, .T. ) ;
#10442=ORIENTED_EDGE ( 'NONE', *, *, #3144, .F. ) ;
#10449=APPLICATION_CONTEXT ( 'automotive_design' ) ;
#10450=CARTESIAN_POINT ( 'NONE',  ( 58.68170757442803165, 39.57655509336063204, 33.00000000000000000 ) ) ;
#10492=VERTEX_POINT ( 'NONE', #9496 ) ;
#10519=PLANE ( 'NONE',  #2164 ) ;
#10536=DIRECTION ( 'NONE',  ( -0.9701425001453319874, -0.2425356250363330801, 0.000000000000000000 ) ) ;
#10577=EDGE_CURVE ( 'NONE', #6772, #1377, #8190, .T. ) ;
#10582=LINE ( 'NONE', #2688, #11790 ) ;
#10583=LINE ( 'NONE', #7128, #5195 ) ;
#10621=ORIENTED_EDGE ( 'NONE', *, *, #4953, .T. ) ;
#10645=AXIS2_PLACEMENT_3D ( 'NONE', #3627, #395, #8357 ) ;
#10668=FILL_AREA_STYLE ('',( #652 ) ) ;
#10674=ORIENTED_EDGE ( 'NONE', *, *, #8702, .T. ) ;
#10681=CARTESIAN_POINT ( 'NONE',  ( 21.68170757442799967, 141.2731697022880155, 33.00000000000000000 ) ) ;
#10686=EDGE_CURVE ( 'NONE', #6772, #14419, #9955, .T. ) ;
#10749=CARTESIAN_POINT ( 'NONE',  ( 95.04167153547044222, -149.6197612287760705, 28.00000000000000000 ) ) ;
#10771=ORIENTED_EDGE ( 'NONE', *, *, #751, .F. ) ;
#10772=CARTESIAN_POINT ( 'NONE',  ( 21.68170757442799967, 141.2731697022880155, -28.00000000000000000 ) ) ;
#10784=CARTESIAN_POINT ( 'NONE',  ( 62.10586122665986863, -20.42344490663937151, -33.00000000000000000 ) ) ;
#10788=EDGE_CURVE ( 'NONE', #6997, #10492, #12572, .T. ) ;
#10829=DIRECTION ( 'NONE',  ( 0.000000000000000000, 0.000000000000000000, 1.000000000000000000 ) ) ;
#10831=FACE_OUTER_BOUND ( 'NONE', #5292, .T. ) ;
#10868=LINE ( 'NONE', #839, #1258 ) ;
#10869=CARTESIAN_POINT ( 'NONE',  ( 95.04167153547044222, -149.6197612287760705, -28.00000000000000000 ) ) ;
#10870=VERTEX_POINT ( 'NONE', #1376 ) ;
#10942=EDGE_LOOP ( 'NONE', ( #12448, #8189, #11760, #81 ) ) ;
#10963=EDGE_CURVE ( 'NONE', #11964, #9506, #1531, .T. ) ;
#10982=AXIS2_PLACEMENT_3D ( 'NONE', #469, #9239, #9313 ) ;
#10987=DIRECTION ( 'NONE',  ( 1.000000000000000000, 1.927470528863118802E-16, 0.000000000000000000 ) ) ;
#11009=CARTESIAN_POINT ( 'NONE',  ( 76.68170757442796059, 3.003422806631532356E-13, -199.4258611313499330 ) ) ;
#11025=AXIS2_PLACEMENT_3D ( 'NONE', #167, #6524, #5441 ) ;
#11062=DIRECTION ( 'NONE',  ( -0.2425356250363330801, 0.9701425001453319874, 0.000000000000000000 ) ) ;
#11078=CARTESIAN_POINT ( 'NONE',  ( 71.80728622811317052, -20.42344490663941414, 28.00000000000000000 ) ) ;
#11092=CARTESIAN_POINT ( 'NONE',  ( 58.68170757442803165, 39.57655509336063204, -33.00000000000000000 ) ) ;
#11158=EDGE_CURVE ( 'NONE', #13026, #4341, #6055, .T. ) ;
#11181=ORIENTED_EDGE ( 'NONE', *, *, #6820, .T. ) ;
#11206=EDGE_CURVE ( 'NONE', #3642, #14419, #6280, .T. ) ;
#11223=STYLED_ITEM ( 'NONE', ( #7426 ), #11635 ) ;
#11226=PRESENTATION_STYLE_ASSIGNMENT (( #12532 ) ) ;
#11272=CARTESIAN_POINT ( 'NONE',  ( 21.68170757442799967, 141.2731697022880155, 33.00000000000000000 ) ) ;
#11299=CARTESIAN_POINT ( 'NONE',  ( 71.80728622811317052, -20.42344490663941414, -28.00000000000000000 ) ) ;
#11329=EDGE_LOOP ( 'NONE', ( #14011, #14039, #9000, #431 ) ) ;
#11341=EDGE_CURVE ( 'NONE', #4128, #6195, #5190, .T. ) ;
#11342=ADVANCED_FACE ( 'NONE', ( #7513 ), #7310, .F. ) ;
#11350=ORIENTED_EDGE ( 'NONE', *, *, #11730, .F. ) ;
#11384=CARTESIAN_POINT ( 'NONE',  ( 0.000000000000000000, -20.42344490663941414, 33.00000000000000000 ) ) ;
#11434=SHAPE_REPRESENTATION_RELATIONSHIP ( 'NONE' , 'NONE' ,  #7389, #4561 ) ;
#11472=CARTESIAN_POINT ( 'NONE',  ( 71.80728622811317052, -17.99808865627608512, -28.00000000000000000 ) ) ;
#11513=DIRECTION ( 'NONE',  ( -0.2425356250363330801, 0.9701425001453319874, 0.000000000000000000 ) ) ;
#11543=ORIENTED_EDGE ( 'NONE', *, *, #3402, .F. ) ;
#11573=CARTESIAN_POINT ( 'NONE',  ( 88.22284556172391490, -83.66032599071898801, -28.00000000000000000 ) ) ;
#11578=PLANE ( 'NONE',  #10982 ) ;
#11598=DIRECTION ( 'NONE',  ( 0.000000000000000000, 0.000000000000000000, 1.000000000000000000 ) ) ;
#11599=ORIENTED_EDGE ( 'NONE', *, *, #917, .F. ) ;
#11602=CARTESIAN_POINT ( 'NONE',  ( 36.31750732272606541, 144.5765550933605823, 33.00000000000000000 ) ) ;
#11633=VERTEX_POINT ( 'NONE', #6196 ) ;
#11635=MANIFOLD_SOLID_BREP ( 'Fillet1', #13918 ) ;
#11663=ORIENTED_EDGE ( 'NONE', *, *, #5466, .F. ) ;
#11678=VECTOR ( 'NONE', #14195, 1000.000000000000000 ) ;
#11729=LINE ( 'NONE', #4918, #774 ) ;
#11730=EDGE_CURVE ( 'NONE', #9429, #1767, #12054, .T. ) ;
#11732=ORIENTED_EDGE ( 'NONE', *, *, #14255, .F. ) ;
#11737=DIRECTION ( 'NONE',  ( 0.000000000000000000, -1.000000000000000000, 0.000000000000000000 ) ) ;
#11743=LINE ( 'NONE', #5938, #10330 ) ;
#11760=ORIENTED_EDGE ( 'NONE', *, *, #13902, .T. ) ;
#11787=PLANE ( 'NONE',  #13849 ) ;
#11790=VECTOR ( 'NONE', #7127, 1000.000000000000000 ) ;
#11796=CARTESIAN_POINT ( 'NONE',  ( 36.31750732272606541, 144.5765550933605823, -33.00000000000000000 ) ) ;
#11810=CARTESIAN_POINT ( 'NONE',  ( 31.38313257588132288, 143.6985259526512948, 33.00000000000000000 ) ) ;
#11839=SURFACE_SIDE_STYLE ('',( #9495 ) ) ;
#11850=DIRECTION ( 'NONE',  ( -1.000000000000000000, 0.000000000000000000, 0.000000000000000000 ) ) ;
#11854=CIRCLE ( 'NONE', #5528, 300.0000000000001137 ) ;
#11865=AXIS2_PLACEMENT_3D ( 'NONE', #10273, #5870, #10356 ) ;
#11910=CARTESIAN_POINT ( 'NONE',  ( 62.10586122665986863, -20.42344490663937151, 33.00000000000000000 ) ) ;
#11933=ADVANCED_FACE ( 'NONE', ( #7344 ), #9475, .F. ) ;
#11949=LINE ( 'NONE', #1780, #7508 ) ;
#11964=VERTEX_POINT ( 'NONE', #11272 ) ;
#11975=ORIENTED_EDGE ( 'NONE', *, *, #3144, .T. ) ;
#11983=( GEOMETRIC_REPRESENTATION_CONTEXT ( 3 ) GLOBAL_UNCERTAINTY_ASSIGNED_CONTEXT ( ( #1784 ) ) GLOBAL_UNIT_ASSIGNED_CONTEXT ( ( #2241, #3487, #42 ) ) REPRESENTATION_CONTEXT ( 'NONE', 'WORKASPACE' ) );
#11989=EDGE_CURVE ( 'NONE', #10870, #9890, #5694, .T. ) ;
#11993=VECTOR ( 'NONE', #5055, 1000.000000000000000 ) ;
#11997=CARTESIAN_POINT ( 'NONE',  ( 0.000000000000000000, -20.42344490663941414, -199.4258611313499330 ) ) ;
#12001=CARTESIAN_POINT ( 'NONE',  ( 76.68170757442801744, 39.57655509336063204, -33.00000000000000000 ) ) ;
#12028=ORIENTED_EDGE ( 'NONE', *, *, #6526, .T. ) ;
#12031=CARTESIAN_POINT ( 'NONE',  ( 95.04167153547044222, -149.6197612287760705, -32.99999999999999289 ) ) ;
#12054=LINE ( 'NONE', #9319, #4483 ) ;
#12064=DIRECTION ( 'NONE',  ( 0.000000000000000000, 0.000000000000000000, -1.000000000000000000 ) ) ;
#12073=EDGE_CURVE ( 'NONE', #4637, #9429, #5492, .T. ) ;
#12118=CARTESIAN_POINT ( 'NONE',  ( 21.68170757442799967, 141.2731697022880155, 28.00000000000000000 ) ) ;
#12302=FACE_OUTER_BOUND ( 'NONE', #764, .T. ) ;
#12317=ORIENTED_EDGE ( 'NONE', *, *, #13904, .F. ) ;
#12330=DIRECTION ( 'NONE',  ( 0.000000000000000000, 0.000000000000000000, 1.000000000000000000 ) ) ;
#12336=ORIENTED_EDGE ( 'NONE', *, *, #11158, .T. ) ;
#12415=ORIENTED_EDGE ( 'NONE', *, *, #11158, .F. ) ;
#12432=VECTOR ( 'NONE', #12330, 1000.000000000000000 ) ;
#12448=ORIENTED_EDGE ( 'NONE', *, *, #11341, .F. ) ;
#12466=VECTOR ( 'NONE', #6789, 1000.000000000000000 ) ;
#12472=DIRECTION ( 'NONE',  ( 0.000000000000000000, 0.000000000000000000, 1.000000000000000000 ) ) ;
#12473=SURFACE_STYLE_FILL_AREA ( #325 ) ;
#12485=ADVANCED_FACE ( 'NONE', ( #1586 ), #10519, .F. ) ;
#12491=DIRECTION ( 'NONE',  ( -0.2425356250363330801, 0.9701425001453319874, 0.000000000000000000 ) ) ;
#12500=PRODUCT_DEFINITION ( 'UNKNOWN', '', #1023, #6739 ) ;
#12531=VECTOR ( 'NONE', #19, 999.9999999999998863 ) ;
#12532=SURFACE_STYLE_USAGE ( .BOTH. , #4719 ) ;
#12554=DIRECTION ( 'NONE',  ( 1.000000000000000000, 0.000000000000000000, 0.000000000000000000 ) ) ;
#12559=VECTOR ( 'NONE', #7843, 999.9999999999998863 ) ;
#12572=LINE ( 'NONE', #4618, #2837 ) ;
#12587=VECTOR ( 'NONE', #7510, 1000.000000000000000 ) ;
#12591=ORIENTED_EDGE ( 'NONE', *, *, #7298, .T. ) ;
#12601=LINE ( 'NONE', #2671, #5983 ) ;
#12657=ORIENTED_EDGE ( 'NONE', *, *, #9421, .F. ) ;
#12667=ORIENTED_EDGE ( 'NONE', *, *, #7934, .T. ) ;
#12762=ADVANCED_FACE ( 'NONE', ( #12302 ), #5417, .F. ) ;
#12802=CARTESIAN_POINT ( 'NONE',  ( 88.22284556172391490, -83.66032599071898801, -28.00000000000000000 ) ) ;
#12809=VECTOR ( 'NONE', #12472, 1000.000000000000000 ) ;
#12832=DIRECTION ( 'NONE',  ( 0.000000000000000000, 0.000000000000000000, 1.000000000000000000 ) ) ;
#12833=LINE ( 'NONE', #6382, #4831 ) ;
#12843=ORIENTED_EDGE ( 'NONE', *, *, #4953, .F. ) ;
#12852=ORIENTED_EDGE ( 'NONE', *, *, #3622, .T. ) ;
#12861=CARTESIAN_POINT ( 'NONE',  ( 76.68170757442801744, 29.57655509336063204, -33.00000000000000000 ) ) ;
#12864=DIRECTION ( 'NONE',  ( -1.000000000000000000, 2.312964634635741951E-14, 0.000000000000000000 ) ) ;
#12918=EDGE_CURVE ( 'NONE', #1783, #9506, #11949, .T. ) ;
#12946=VECTOR ( 'NONE', #7171, 999.9999999999998863 ) ;
#12961=DIRECTION ( 'NONE',  ( 0.000000000000000000, 0.000000000000000000, 1.000000000000000000 ) ) ;
#12970=CARTESIAN_POINT ( 'NONE',  ( 62.10586122665989706, -20.42344490663939993, -28.00000000000000000 ) ) ;
#12975=ORIENTED_EDGE ( 'NONE', *, *, #4352, .F. ) ;
#12989=ORIENTED_EDGE ( 'NONE', *, *, #10400, .F. ) ;
#12999=AXIS2_PLACEMENT_3D ( 'NONE', #5654, #10131, #116 ) ;
#13003=DIRECTION ( 'NONE',  ( 0.9701425001453319874, 0.2425356250363330801, 0.000000000000000000 ) ) ;
#13026=VERTEX_POINT ( 'NONE', #13342 ) ;
#13072=ORIENTED_EDGE ( 'NONE', *, *, #3622, .F. ) ;
#13102=FACE_OUTER_BOUND ( 'NONE', #4640, .T. ) ;
#13104=EDGE_CURVE ( 'NONE', #8097, #6195, #3174, .T. ) ;
#13115=EDGE_LOOP ( 'NONE', ( #4655, #9152, #4985, #8220 ) ) ;
#13175=LINE ( 'NONE', #5391, #1252 ) ;
#13222=ORIENTED_EDGE ( 'NONE', *, *, #4361, .T. ) ;
#13229=VERTEX_POINT ( 'NONE', #7011 ) ;
#13304=ORIENTED_EDGE ( 'NONE', *, *, #5849, .F. ) ;
#13310=DIRECTION ( 'NONE',  ( 0.9701425001453319874, 0.2425356250363330801, 0.000000000000000000 ) ) ;
#13334=ORIENTED_EDGE ( 'NONE', *, *, #13104, .F. ) ;
#13342=CARTESIAN_POINT ( 'NONE',  ( 76.68170757442801744, 144.5765550933605823, -33.00000000000000000 ) ) ;
#13351=DIRECTION ( 'NONE',  ( 1.000000000000000000, 0.000000000000000000, 0.000000000000000000 ) ) ;
#13356=AXIS2_PLACEMENT_3D ( 'NONE', #1664, #6113, #12864 ) ;
#13374=DIRECTION ( 'NONE',  ( 0.000000000000000000, -1.000000000000000000, 0.000000000000000000 ) ) ;
#13411=CARTESIAN_POINT ( 'NONE',  ( 31.41872415839353039, 143.5561596226024790, 28.00000000000000000 ) ) ;
#13427=DIRECTION ( 'NONE',  ( 1.000000000000000000, 1.927470528863118802E-16, 0.000000000000000000 ) ) ;
#13470=ORIENTED_EDGE ( 'NONE', *, *, #118, .T. ) ;
#13481=DIRECTION ( 'NONE',  ( 1.927470528863118802E-16, -1.000000000000000000, -0.000000000000000000 ) ) ;
#13581=MECHANICAL_DESIGN_GEOMETRIC_PRESENTATION_REPRESENTATION('',(#11223),#487);
#13614=CARTESIAN_POINT ( 'NONE',  ( 58.68170757442803165, 34.50422595846454499, -28.00000000000000000 ) ) ;
#13626=DIRECTION ( 'NONE',  ( 3.916739600140467622E-15, -1.000000000000000000, -0.000000000000000000 ) ) ;
#13630=CARTESIAN_POINT ( 'NONE',  ( 36.31750732272606541, 144.5765550933605823, -33.00000000000000000 ) ) ;
#13647=ADVANCED_FACE ( 'NONE', ( #7121 ), #7413, .T. ) ;
#13650=AXIS2_PLACEMENT_3D ( 'NONE', #8788, #2143, #11062 ) ;
#13672=VERTEX_POINT ( 'NONE', #14312 ) ;
#13753=VECTOR ( 'NONE', #14268, 1000.000000000000000 ) ;
#13818=CARTESIAN_POINT ( 'NONE',  ( 76.68170757442801744, 29.57655509336063204, 33.00000000000000000 ) ) ;
#13830=DIRECTION ( 'NONE',  ( 0.000000000000000000, 0.000000000000000000, -1.000000000000000000 ) ) ;
#13833=ORIENTED_EDGE ( 'NONE', *, *, #9421, .T. ) ;
#13849=AXIS2_PLACEMENT_3D ( 'NONE', #12802, #10536, #733 ) ;
#13868=VERTEX_POINT ( 'NONE', #170 ) ;
#13885=VERTEX_POINT ( 'NONE', #3340 ) ;
#13902=EDGE_CURVE ( 'NONE', #7846, #10355, #11729, .T. ) ;
#13904=EDGE_CURVE ( 'NONE', #13229, #8393, #3757, .T. ) ;
#13918=CLOSED_SHELL ( 'NONE', ( #5172, #5082, #10161, #12485, #5768, #13647, #14348, #2253, #5993, #14263, #5429, #11933, #5500, #2691, #8475, #12762, #4488, #11342, #3541 ) ) ;
#13937=EDGE_LOOP ( 'NONE', ( #2951, #11975, #1502, #10359 ) ) ;
#14011=ORIENTED_EDGE ( 'NONE', *, *, #10303, .T. ) ;
#14016=LINE ( 'NONE', #8351, #9983 ) ;
#14039=ORIENTED_EDGE ( 'NONE', *, *, #1535, .T. ) ;
#14116=FACE_OUTER_BOUND ( 'NONE', #13115, .T. ) ;
#14163=ORIENTED_EDGE ( 'NONE', *, *, #10431, .T. ) ;
#14181=DIRECTION ( 'NONE',  ( -1.000000000000000000, 0.000000000000000000, 0.000000000000000000 ) ) ;
#14195=DIRECTION ( 'NONE',  ( -3.916739600140467622E-15, 1.000000000000000000, 0.000000000000000000 ) ) ;
#14214=CARTESIAN_POINT ( 'NONE',  ( 22.28098402457126426, 141.4229888148238103, 1.219362754841566419E-12 ) ) ;
#14230=VECTOR ( 'NONE', #1517, 1000.000000000000000 ) ;
#14233=AXIS2_PLACEMENT_3D ( 'NONE', #11009, #2992, #2171 ) ;
#14242=ORIENTED_EDGE ( 'NONE', *, *, #3901, .T. ) ;
#14255=EDGE_CURVE ( 'NONE', #6248, #687, #6737, .T. ) ;
#14263=ADVANCED_FACE ( 'NONE', ( #4353 ), #5498, .F. ) ;
#14266=LINE ( 'NONE', #3011, #12587 ) ;
#14268=DIRECTION ( 'NONE',  ( -1.000000000000000000, 0.000000000000000000, 0.000000000000000000 ) ) ;
#14312=CARTESIAN_POINT ( 'NONE',  ( 22.28098402457051463, 141.4229888148235830, -32.99999999999999289 ) ) ;
#14348=ADVANCED_FACE ( 'NONE', ( #259 ), #9248, .T. ) ;
#14356=DIRECTION ( 'NONE',  ( 0.000000000000000000, 0.000000000000000000, 1.000000000000000000 ) ) ;
#14368=CARTESIAN_POINT ( 'NONE',  ( 76.68170757442801744, 29.57655509336063204, 33.00000000000000000 ) ) ;
#14373=CARTESIAN_POINT ( 'NONE',  ( 62.10586122665986863, -20.42344490663941414, -27.99999999999999645 ) ) ;
#14385=DIRECTION ( 'NONE',  ( 0.000000000000000000, 1.000000000000000000, 0.000000000000000000 ) ) ;
#14419=VERTEX_POINT ( 'NONE', #9620 ) ;
#14444=CARTESIAN_POINT ( 'NONE',  ( 58.68170757442803165, 29.57655509336062849, 33.00000000000000000 ) ) ;
#14456=LINE ( 'NONE', #5518, #7555 ) ;
ENDSEC;
END-ISO-10303-21;
